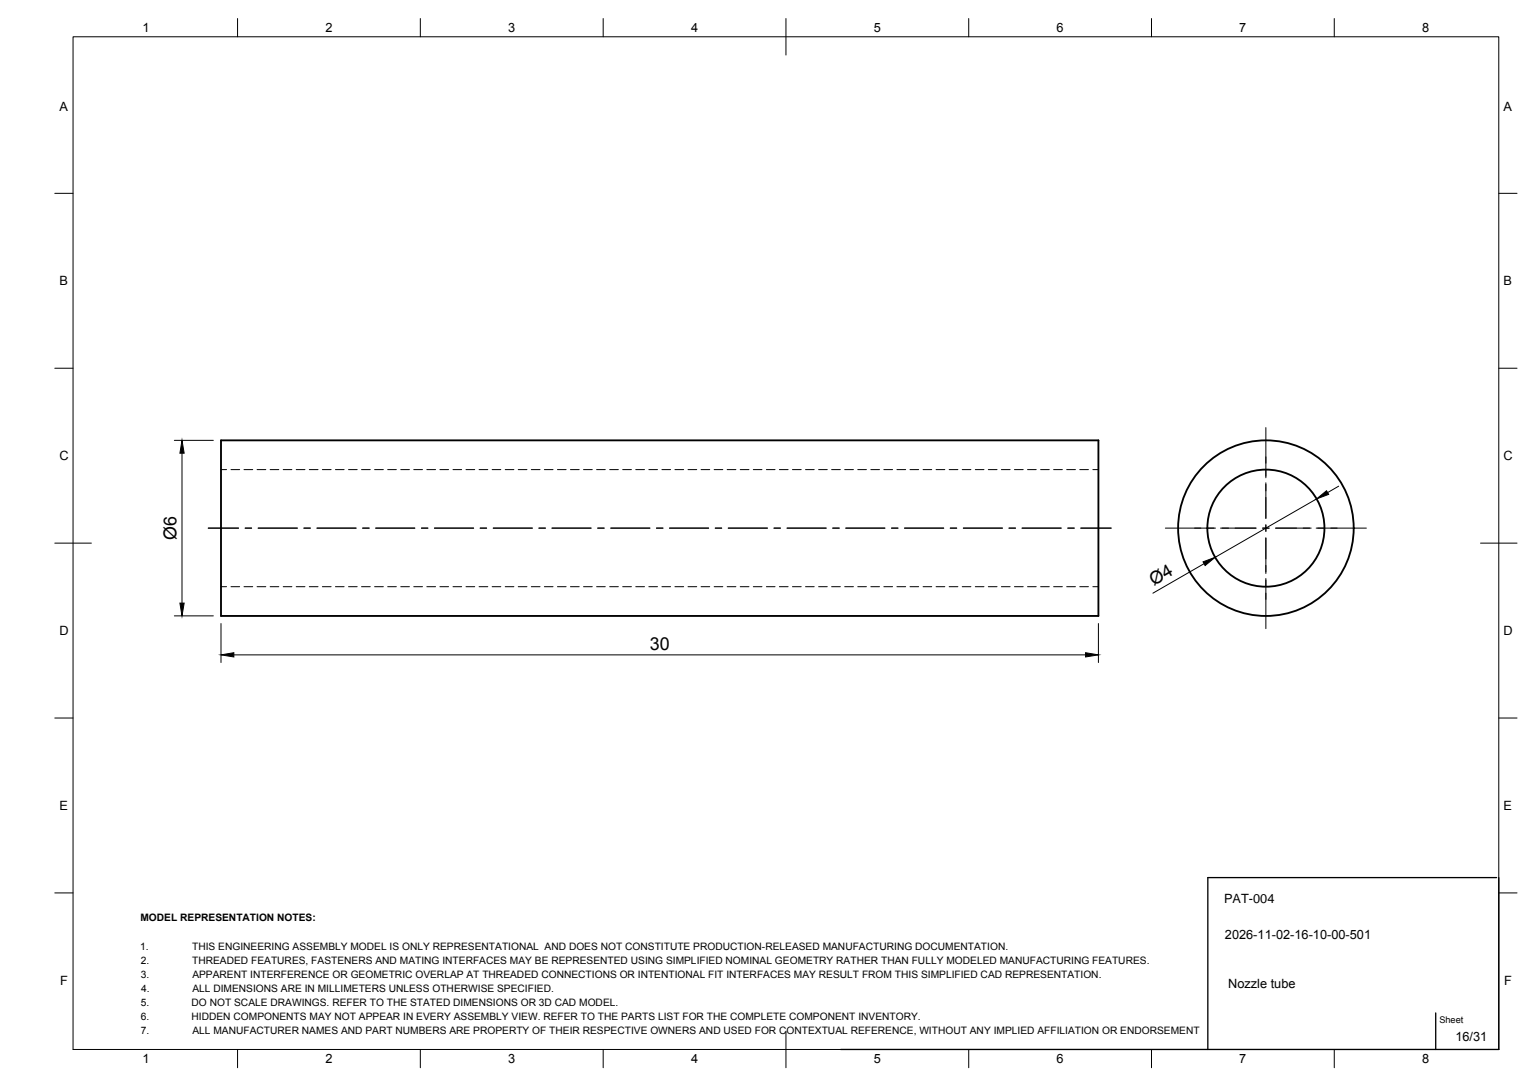
ISO-10303-21;
HEADER;
/* Generated by software containing ST-Developer
 * from STEP Tools, Inc. (www.steptools.com) 
 */

FILE_DESCRIPTION(
/* description */ ('Air blow-off nozzle station'),
/* implementation_level */ '2;1');

FILE_NAME(
/* name */ 'Nozzle tube.step',
/* time_stamp */ '2026-10-27T10:53:54-07:00',
/* author */ (''),
/* organization */ (''),
/* preprocessor_version */ 'ST-DEVELOPER v20.2',
/* originating_system */ 'Autodesk Translation Framework v15.17.0.0',
/* authorisation */ '');

FILE_SCHEMA (('AUTOMOTIVE_DESIGN { 1 0 10303 214 3 1 1 }'));
ENDSEC;

DATA;
#10=MECHANICAL_DESIGN_GEOMETRIC_PRESENTATION_REPRESENTATION('',(#252),#7897);
#202=SHAPE_REPRESENTATION_RELATIONSHIP('SRR','None',#8017,#227);
#227=ADVANCED_BREP_SHAPE_REPRESENTATION('',(#275),#7884);
#252=STYLED_ITEM('',(#8206),#275);
#275=MANIFOLD_SOLID_BREP('Body1',#4303);
#339=FACE_BOUND('',#1044,.T.);
#340=FACE_BOUND('',#1046,.T.);
#506=PLANE('',#4923);
#507=PLANE('',#4924);
#731=FACE_OUTER_BOUND('',#1041,.T.);
#732=FACE_OUTER_BOUND('',#1042,.T.);
#733=FACE_OUTER_BOUND('',#1043,.T.);
#734=FACE_OUTER_BOUND('',#1045,.T.);
#1041=EDGE_LOOP('',(#3745,#3746,#3747,#3748));
#1042=EDGE_LOOP('',(#3749,#3750,#3751,#3752));
#1043=EDGE_LOOP('',(#3753));
#1044=EDGE_LOOP('',(#3754));
#1045=EDGE_LOOP('',(#3755));
#1046=EDGE_LOOP('',(#3756));
#1445=LINE('',#7562,#1799);
#1446=LINE('',#7568,#1800);
#1799=VECTOR('',#6039,0.2);
#1800=VECTOR('',#6046,0.3);
#1947=CIRCLE('',#4918,0.2);
#1948=CIRCLE('',#4919,0.2);
#1949=CIRCLE('',#4921,0.3);
#1950=CIRCLE('',#4922,0.3);
#2292=VERTEX_POINT('',#7559);
#2293=VERTEX_POINT('',#7561);
#2294=VERTEX_POINT('',#7565);
#2295=VERTEX_POINT('',#7567);
#2790=EDGE_CURVE('',#2292,#2292,#1947,.T.);
#2791=EDGE_CURVE('',#2292,#2293,#1445,.T.);
#2792=EDGE_CURVE('',#2293,#2293,#1948,.T.);
#2793=EDGE_CURVE('',#2294,#2294,#1949,.T.);
#2794=EDGE_CURVE('',#2294,#2295,#1446,.T.);
#2795=EDGE_CURVE('',#2295,#2295,#1950,.T.);
#3745=ORIENTED_EDGE('',*,*,#2790,.F.);
#3746=ORIENTED_EDGE('',*,*,#2791,.T.);
#3747=ORIENTED_EDGE('',*,*,#2792,.T.);
#3748=ORIENTED_EDGE('',*,*,#2791,.F.);
#3749=ORIENTED_EDGE('',*,*,#2793,.F.);
#3750=ORIENTED_EDGE('',*,*,#2794,.T.);
#3751=ORIENTED_EDGE('',*,*,#2795,.T.);
#3752=ORIENTED_EDGE('',*,*,#2794,.F.);
#3753=ORIENTED_EDGE('',*,*,#2793,.T.);
#3754=ORIENTED_EDGE('',*,*,#2790,.T.);
#3755=ORIENTED_EDGE('',*,*,#2795,.F.);
#3756=ORIENTED_EDGE('',*,*,#2792,.F.);
#4001=CYLINDRICAL_SURFACE('',#4917,0.2);
#4002=CYLINDRICAL_SURFACE('',#4920,0.3);
#4221=ADVANCED_FACE('',(#731),#4001,.F.);
#4222=ADVANCED_FACE('',(#732),#4002,.T.);
#4223=ADVANCED_FACE('',(#733,#339),#506,.T.);
#4224=ADVANCED_FACE('',(#734,#340),#507,.F.);
#4303=CLOSED_SHELL('',(#4221,#4222,#4223,#4224));
#4916=AXIS2_PLACEMENT_3D('',#7557,#6033,#6034);
#4917=AXIS2_PLACEMENT_3D('',#7558,#6035,#6036);
#4918=AXIS2_PLACEMENT_3D('',#7560,#6037,#6038);
#4919=AXIS2_PLACEMENT_3D('',#7563,#6040,#6041);
#4920=AXIS2_PLACEMENT_3D('',#7564,#6042,#6043);
#4921=AXIS2_PLACEMENT_3D('',#7566,#6044,#6045);
#4922=AXIS2_PLACEMENT_3D('',#7569,#6047,#6048);
#4923=AXIS2_PLACEMENT_3D('',#7570,#6049,#6050);
#4924=AXIS2_PLACEMENT_3D('',#7571,#6051,#6052);
#6033=DIRECTION('axis',(0.,0.,1.));
#6034=DIRECTION('refdir',(1.,0.,0.));
#6035=DIRECTION('center_axis',(0.,1.,0.));
#6036=DIRECTION('ref_axis',(1.,0.,0.));
#6037=DIRECTION('center_axis',(0.,-1.,0.));
#6038=DIRECTION('ref_axis',(1.,0.,0.));
#6039=DIRECTION('',(0.,-1.,0.));
#6040=DIRECTION('center_axis',(0.,-1.,0.));
#6041=DIRECTION('ref_axis',(1.,0.,0.));
#6042=DIRECTION('center_axis',(0.,1.,0.));
#6043=DIRECTION('ref_axis',(1.,0.,0.));
#6044=DIRECTION('center_axis',(0.,1.,0.));
#6045=DIRECTION('ref_axis',(1.,0.,0.));
#6046=DIRECTION('',(0.,-1.,0.));
#6047=DIRECTION('center_axis',(0.,1.,0.));
#6048=DIRECTION('ref_axis',(1.,0.,0.));
#6049=DIRECTION('center_axis',(0.,1.,0.));
#6050=DIRECTION('ref_axis',(1.,0.,0.));
#6051=DIRECTION('center_axis',(0.,1.,0.));
#6052=DIRECTION('ref_axis',(1.,0.,0.));
#7557=CARTESIAN_POINT('',(0.,0.,0.));
#7558=CARTESIAN_POINT('Origin',(-3.,-7.2,23.));
#7559=CARTESIAN_POINT('',(-3.2,-4.2,23.));
#7560=CARTESIAN_POINT('Origin',(-3.,-4.2,23.));
#7561=CARTESIAN_POINT('',(-3.2,-7.2,23.));
#7562=CARTESIAN_POINT('',(-3.2,-7.2,23.));
#7563=CARTESIAN_POINT('Origin',(-3.,-7.2,23.));
#7564=CARTESIAN_POINT('Origin',(-3.,-7.2,23.));
#7565=CARTESIAN_POINT('',(-3.3,-4.2,23.));
#7566=CARTESIAN_POINT('Origin',(-3.,-4.2,23.));
#7567=CARTESIAN_POINT('',(-3.3,-7.2,23.));
#7568=CARTESIAN_POINT('',(-3.3,-7.2,23.));
#7569=CARTESIAN_POINT('Origin',(-3.,-7.2,23.));
#7570=CARTESIAN_POINT('Origin',(-3.,-4.2,23.));
#7571=CARTESIAN_POINT('Origin',(-3.,-7.2,23.));
#7852=UNCERTAINTY_MEASURE_WITH_UNIT(LENGTH_MEASURE(0.001),#7898,
'DISTANCE_ACCURACY_VALUE',
'Maximum model space distance between geometric entities at asserted c
onnectivities');
#7865=UNCERTAINTY_MEASURE_WITH_UNIT(LENGTH_MEASURE(0.001),#7898,
'DISTANCE_ACCURACY_VALUE',
'Maximum model space distance between geometric entities at asserted c
onnectivities');
#7884=(
GEOMETRIC_REPRESENTATION_CONTEXT(3)
GLOBAL_UNCERTAINTY_ASSIGNED_CONTEXT((#7852))
GLOBAL_UNIT_ASSIGNED_CONTEXT((#7898,#7900,#7901))
REPRESENTATION_CONTEXT('','3D')
);
#7897=(
GEOMETRIC_REPRESENTATION_CONTEXT(3)
GLOBAL_UNCERTAINTY_ASSIGNED_CONTEXT((#7865))
GLOBAL_UNIT_ASSIGNED_CONTEXT((#7898,#7900,#7901))
REPRESENTATION_CONTEXT('','3D')
);
#7898=(
LENGTH_UNIT()
NAMED_UNIT(*)
SI_UNIT(.CENTI.,.METRE.)
);
#7900=(
NAMED_UNIT(*)
PLANE_ANGLE_UNIT()
SI_UNIT($,.RADIAN.)
);
#7901=(
NAMED_UNIT(*)
SI_UNIT($,.STERADIAN.)
SOLID_ANGLE_UNIT()
);
#7920=SHAPE_DEFINITION_REPRESENTATION(#7968,#8017);
#7968=PRODUCT_DEFINITION_SHAPE('',$,#8049);
#8017=SHAPE_REPRESENTATION('',(#4916),#7884);
#8030=PRODUCT_DEFINITION_CONTEXT('part definition',#8125,'design');
#8049=PRODUCT_DEFINITION('Nozzle tube','Nozzle tube',#8080,#8030);
#8080=PRODUCT_DEFINITION_FORMATION('',$,#8145);
#8125=APPLICATION_CONTEXT(
'Core Data for Automotive Mechanical Design Process');
#8126=PRODUCT_CONTEXT('part definition',#8125,'mechanical');
#8145=PRODUCT('Nozzle tube','Nozzle tube','Nozzle tube',(#8126));
#8200=COLOUR_RGB('Light Blue',0.38,0.62,0.78);
#8201=FILL_AREA_STYLE_COLOUR('',#8200);
#8202=FILL_AREA_STYLE('',(#8201));
#8203=SURFACE_STYLE_FILL_AREA(#8202);
#8204=SURFACE_SIDE_STYLE('',(#8203));
#8205=SURFACE_STYLE_USAGE(.BOTH.,#8204);
#8206=PRESENTATION_STYLE_ASSIGNMENT((#8205));
ENDSEC;
END-ISO-10303-21;
